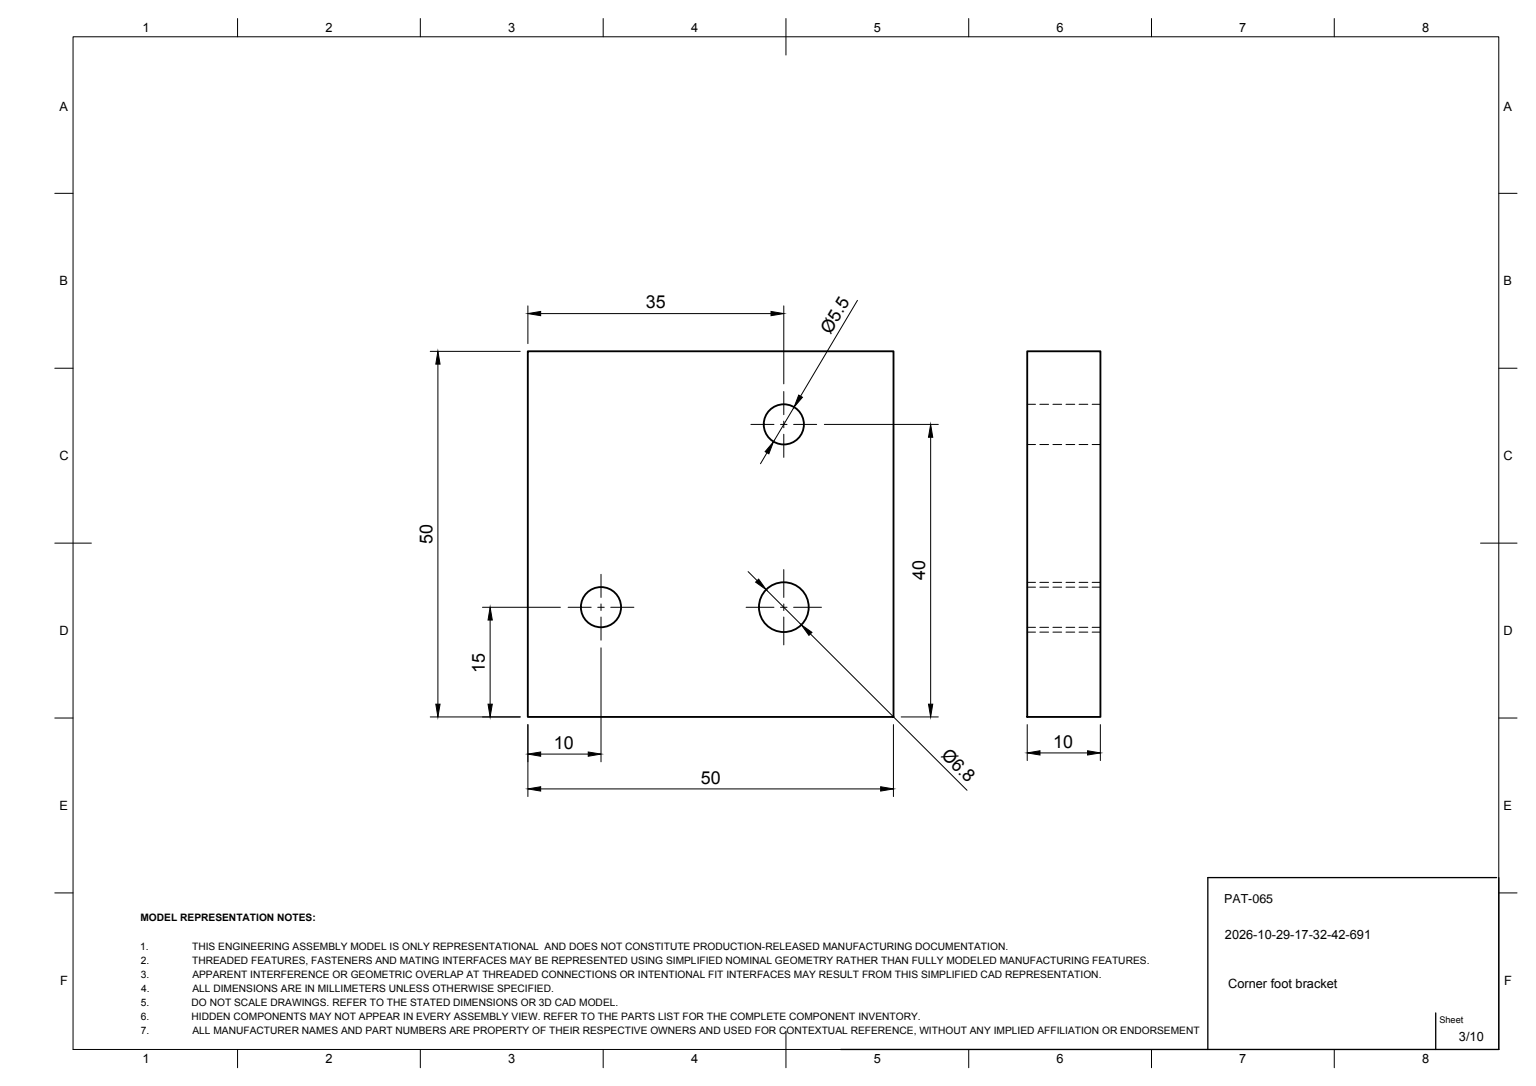
ISO-10303-21;
HEADER;
/* Generated by software containing ST-Developer
 * from STEP Tools, Inc. (www.steptools.com) 
 */

FILE_DESCRIPTION(
/* description */ ('PAT-065'),
/* implementation_level */ '2;1');

FILE_NAME(
/* name */ 'Corner foot bracket.step',
/* time_stamp */ '2026-10-28T22:09:22-07:00',
/* author */ (''),
/* organization */ (''),
/* preprocessor_version */ 'ST-DEVELOPER v20.2',
/* originating_system */ 'Autodesk Translation Framework v15.17.0.0',
/* authorisation */ '');

FILE_SCHEMA (('AUTOMOTIVE_DESIGN { 1 0 10303 214 3 1 1 }'));
ENDSEC;

DATA;
#10=MECHANICAL_DESIGN_GEOMETRIC_PRESENTATION_REPRESENTATION('',(#158),#5502);
#138=SHAPE_REPRESENTATION_RELATIONSHIP('SRR','None',#5555,#148);
#148=ADVANCED_BREP_SHAPE_REPRESENTATION('',(#168),#5491);
#158=STYLED_ITEM('',(#5673),#168);
#168=MANIFOLD_SOLID_BREP('Body1',#3205);
#177=FACE_BOUND('',#519,.T.);
#178=FACE_BOUND('',#520,.T.);
#179=FACE_BOUND('',#521,.T.);
#180=FACE_BOUND('',#523,.T.);
#181=FACE_BOUND('',#524,.T.);
#182=FACE_BOUND('',#525,.T.);
#201=PLANE('',#3338);
#202=PLANE('',#3339);
#203=PLANE('',#3340);
#204=PLANE('',#3341);
#205=PLANE('',#3342);
#206=PLANE('',#3343);
#337=FACE_OUTER_BOUND('',#511,.T.);
#338=FACE_OUTER_BOUND('',#512,.T.);
#339=FACE_OUTER_BOUND('',#513,.T.);
#340=FACE_OUTER_BOUND('',#514,.T.);
#341=FACE_OUTER_BOUND('',#515,.T.);
#342=FACE_OUTER_BOUND('',#516,.T.);
#343=FACE_OUTER_BOUND('',#517,.T.);
#344=FACE_OUTER_BOUND('',#518,.T.);
#345=FACE_OUTER_BOUND('',#522,.T.);
#511=EDGE_LOOP('',(#2152,#2153,#2154,#2155));
#512=EDGE_LOOP('',(#2156,#2157,#2158,#2159));
#513=EDGE_LOOP('',(#2160,#2161,#2162,#2163));
#514=EDGE_LOOP('',(#2164,#2165,#2166,#2167));
#515=EDGE_LOOP('',(#2168,#2169,#2170,#2171));
#516=EDGE_LOOP('',(#2172,#2173,#2174,#2175));
#517=EDGE_LOOP('',(#2176,#2177,#2178,#2179));
#518=EDGE_LOOP('',(#2180,#2181,#2182,#2183));
#519=EDGE_LOOP('',(#2184));
#520=EDGE_LOOP('',(#2185));
#521=EDGE_LOOP('',(#2186));
#522=EDGE_LOOP('',(#2187,#2188,#2189,#2190));
#523=EDGE_LOOP('',(#2191));
#524=EDGE_LOOP('',(#2192));
#525=EDGE_LOOP('',(#2193));
#709=LINE('',#4537,#1040);
#710=LINE('',#4543,#1041);
#711=LINE('',#4549,#1042);
#712=LINE('',#4554,#1043);
#713=LINE('',#4556,#1044);
#714=LINE('',#4558,#1045);
#715=LINE('',#4559,#1046);
#716=LINE('',#4562,#1047);
#717=LINE('',#4564,#1048);
#718=LINE('',#4565,#1049);
#719=LINE('',#4568,#1050);
#720=LINE('',#4570,#1051);
#721=LINE('',#4571,#1052);
#722=LINE('',#4573,#1053);
#723=LINE('',#4574,#1054);
#1040=VECTOR('',#3626,0.275);
#1041=VECTOR('',#3633,0.275);
#1042=VECTOR('',#3640,0.34);
#1043=VECTOR('',#3645,1.);
#1044=VECTOR('',#3646,1.);
#1045=VECTOR('',#3647,1.);
#1046=VECTOR('',#3648,1.);
#1047=VECTOR('',#3651,1.);
#1048=VECTOR('',#3652,1.);
#1049=VECTOR('',#3653,1.);
#1050=VECTOR('',#3656,1.);
#1051=VECTOR('',#3657,1.);
#1052=VECTOR('',#3658,1.);
#1053=VECTOR('',#3661,1.);
#1054=VECTOR('',#3662,1.);
#1371=CIRCLE('',#3330,0.275);
#1372=CIRCLE('',#3331,0.275);
#1373=CIRCLE('',#3333,0.275);
#1374=CIRCLE('',#3334,0.275);
#1375=CIRCLE('',#3336,0.34);
#1376=CIRCLE('',#3337,0.34);
#1444=VERTEX_POINT('',#4534);
#1445=VERTEX_POINT('',#4536);
#1446=VERTEX_POINT('',#4540);
#1447=VERTEX_POINT('',#4542);
#1448=VERTEX_POINT('',#4546);
#1449=VERTEX_POINT('',#4548);
#1450=VERTEX_POINT('',#4552);
#1451=VERTEX_POINT('',#4553);
#1452=VERTEX_POINT('',#4555);
#1453=VERTEX_POINT('',#4557);
#1454=VERTEX_POINT('',#4561);
#1455=VERTEX_POINT('',#4563);
#1456=VERTEX_POINT('',#4567);
#1457=VERTEX_POINT('',#4569);
#1726=EDGE_CURVE('',#1444,#1444,#1371,.T.);
#1727=EDGE_CURVE('',#1444,#1445,#709,.T.);
#1728=EDGE_CURVE('',#1445,#1445,#1372,.T.);
#1729=EDGE_CURVE('',#1446,#1446,#1373,.T.);
#1730=EDGE_CURVE('',#1446,#1447,#710,.T.);
#1731=EDGE_CURVE('',#1447,#1447,#1374,.T.);
#1732=EDGE_CURVE('',#1448,#1448,#1375,.T.);
#1733=EDGE_CURVE('',#1448,#1449,#711,.T.);
#1734=EDGE_CURVE('',#1449,#1449,#1376,.T.);
#1735=EDGE_CURVE('',#1450,#1451,#712,.T.);
#1736=EDGE_CURVE('',#1451,#1452,#713,.T.);
#1737=EDGE_CURVE('',#1453,#1452,#714,.T.);
#1738=EDGE_CURVE('',#1450,#1453,#715,.T.);
#1739=EDGE_CURVE('',#1454,#1450,#716,.T.);
#1740=EDGE_CURVE('',#1455,#1453,#717,.T.);
#1741=EDGE_CURVE('',#1454,#1455,#718,.T.);
#1742=EDGE_CURVE('',#1456,#1454,#719,.T.);
#1743=EDGE_CURVE('',#1457,#1455,#720,.T.);
#1744=EDGE_CURVE('',#1456,#1457,#721,.T.);
#1745=EDGE_CURVE('',#1451,#1456,#722,.T.);
#1746=EDGE_CURVE('',#1452,#1457,#723,.T.);
#2152=ORIENTED_EDGE('',*,*,#1726,.F.);
#2153=ORIENTED_EDGE('',*,*,#1727,.T.);
#2154=ORIENTED_EDGE('',*,*,#1728,.F.);
#2155=ORIENTED_EDGE('',*,*,#1727,.F.);
#2156=ORIENTED_EDGE('',*,*,#1729,.F.);
#2157=ORIENTED_EDGE('',*,*,#1730,.T.);
#2158=ORIENTED_EDGE('',*,*,#1731,.F.);
#2159=ORIENTED_EDGE('',*,*,#1730,.F.);
#2160=ORIENTED_EDGE('',*,*,#1732,.F.);
#2161=ORIENTED_EDGE('',*,*,#1733,.T.);
#2162=ORIENTED_EDGE('',*,*,#1734,.F.);
#2163=ORIENTED_EDGE('',*,*,#1733,.F.);
#2164=ORIENTED_EDGE('',*,*,#1735,.T.);
#2165=ORIENTED_EDGE('',*,*,#1736,.T.);
#2166=ORIENTED_EDGE('',*,*,#1737,.F.);
#2167=ORIENTED_EDGE('',*,*,#1738,.F.);
#2168=ORIENTED_EDGE('',*,*,#1739,.T.);
#2169=ORIENTED_EDGE('',*,*,#1738,.T.);
#2170=ORIENTED_EDGE('',*,*,#1740,.F.);
#2171=ORIENTED_EDGE('',*,*,#1741,.F.);
#2172=ORIENTED_EDGE('',*,*,#1742,.T.);
#2173=ORIENTED_EDGE('',*,*,#1741,.T.);
#2174=ORIENTED_EDGE('',*,*,#1743,.F.);
#2175=ORIENTED_EDGE('',*,*,#1744,.F.);
#2176=ORIENTED_EDGE('',*,*,#1745,.T.);
#2177=ORIENTED_EDGE('',*,*,#1744,.T.);
#2178=ORIENTED_EDGE('',*,*,#1746,.F.);
#2179=ORIENTED_EDGE('',*,*,#1736,.F.);
#2180=ORIENTED_EDGE('',*,*,#1746,.T.);
#2181=ORIENTED_EDGE('',*,*,#1743,.T.);
#2182=ORIENTED_EDGE('',*,*,#1740,.T.);
#2183=ORIENTED_EDGE('',*,*,#1737,.T.);
#2184=ORIENTED_EDGE('',*,*,#1728,.T.);
#2185=ORIENTED_EDGE('',*,*,#1731,.T.);
#2186=ORIENTED_EDGE('',*,*,#1734,.T.);
#2187=ORIENTED_EDGE('',*,*,#1745,.F.);
#2188=ORIENTED_EDGE('',*,*,#1735,.F.);
#2189=ORIENTED_EDGE('',*,*,#1739,.F.);
#2190=ORIENTED_EDGE('',*,*,#1742,.F.);
#2191=ORIENTED_EDGE('',*,*,#1726,.T.);
#2192=ORIENTED_EDGE('',*,*,#1729,.T.);
#2193=ORIENTED_EDGE('',*,*,#1732,.T.);
#3004=CYLINDRICAL_SURFACE('',#3329,0.275);
#3005=CYLINDRICAL_SURFACE('',#3332,0.275);
#3006=CYLINDRICAL_SURFACE('',#3335,0.34);
#3031=ADVANCED_FACE('',(#337),#3004,.F.);
#3032=ADVANCED_FACE('',(#338),#3005,.F.);
#3033=ADVANCED_FACE('',(#339),#3006,.F.);
#3034=ADVANCED_FACE('',(#340),#201,.T.);
#3035=ADVANCED_FACE('',(#341),#202,.T.);
#3036=ADVANCED_FACE('',(#342),#203,.T.);
#3037=ADVANCED_FACE('',(#343),#204,.T.);
#3038=ADVANCED_FACE('',(#344,#177,#178,#179),#205,.T.);
#3039=ADVANCED_FACE('',(#345,#180,#181,#182),#206,.F.);
#3205=CLOSED_SHELL('',(#3031,#3032,#3033,#3034,#3035,#3036,#3037,#3038,
#3039));
#3328=AXIS2_PLACEMENT_3D('',#4532,#3620,#3621);
#3329=AXIS2_PLACEMENT_3D('',#4533,#3622,#3623);
#3330=AXIS2_PLACEMENT_3D('',#4535,#3624,#3625);
#3331=AXIS2_PLACEMENT_3D('',#4538,#3627,#3628);
#3332=AXIS2_PLACEMENT_3D('',#4539,#3629,#3630);
#3333=AXIS2_PLACEMENT_3D('',#4541,#3631,#3632);
#3334=AXIS2_PLACEMENT_3D('',#4544,#3634,#3635);
#3335=AXIS2_PLACEMENT_3D('',#4545,#3636,#3637);
#3336=AXIS2_PLACEMENT_3D('',#4547,#3638,#3639);
#3337=AXIS2_PLACEMENT_3D('',#4550,#3641,#3642);
#3338=AXIS2_PLACEMENT_3D('',#4551,#3643,#3644);
#3339=AXIS2_PLACEMENT_3D('',#4560,#3649,#3650);
#3340=AXIS2_PLACEMENT_3D('',#4566,#3654,#3655);
#3341=AXIS2_PLACEMENT_3D('',#4572,#3659,#3660);
#3342=AXIS2_PLACEMENT_3D('',#4575,#3663,#3664);
#3343=AXIS2_PLACEMENT_3D('',#4576,#3665,#3666);
#3620=DIRECTION('axis',(0.,0.,1.));
#3621=DIRECTION('refdir',(1.,0.,0.));
#3622=DIRECTION('center_axis',(0.,0.,1.));
#3623=DIRECTION('ref_axis',(1.,0.,0.));
#3624=DIRECTION('center_axis',(0.,0.,1.));
#3625=DIRECTION('ref_axis',(1.,0.,0.));
#3626=DIRECTION('',(0.,0.,1.));
#3627=DIRECTION('center_axis',(0.,0.,-1.));
#3628=DIRECTION('ref_axis',(1.,0.,0.));
#3629=DIRECTION('center_axis',(0.,0.,1.));
#3630=DIRECTION('ref_axis',(1.,0.,0.));
#3631=DIRECTION('center_axis',(0.,0.,1.));
#3632=DIRECTION('ref_axis',(1.,0.,0.));
#3633=DIRECTION('',(0.,0.,1.));
#3634=DIRECTION('center_axis',(0.,0.,-1.));
#3635=DIRECTION('ref_axis',(1.,0.,0.));
#3636=DIRECTION('center_axis',(0.,0.,1.));
#3637=DIRECTION('ref_axis',(1.,0.,0.));
#3638=DIRECTION('center_axis',(0.,0.,1.));
#3639=DIRECTION('ref_axis',(1.,0.,0.));
#3640=DIRECTION('',(0.,0.,1.));
#3641=DIRECTION('center_axis',(0.,0.,-1.));
#3642=DIRECTION('ref_axis',(1.,0.,0.));
#3643=DIRECTION('center_axis',(0.,1.,0.));
#3644=DIRECTION('ref_axis',(-1.,0.,0.));
#3645=DIRECTION('',(-1.,0.,0.));
#3646=DIRECTION('',(0.,0.,1.));
#3647=DIRECTION('',(-1.,0.,0.));
#3648=DIRECTION('',(0.,0.,1.));
#3649=DIRECTION('center_axis',(1.,0.,0.));
#3650=DIRECTION('ref_axis',(0.,1.,0.));
#3651=DIRECTION('',(0.,1.,0.));
#3652=DIRECTION('',(0.,1.,0.));
#3653=DIRECTION('',(0.,0.,1.));
#3654=DIRECTION('center_axis',(0.,-1.,0.));
#3655=DIRECTION('ref_axis',(1.,0.,0.));
#3656=DIRECTION('',(1.,0.,0.));
#3657=DIRECTION('',(1.,0.,0.));
#3658=DIRECTION('',(0.,0.,1.));
#3659=DIRECTION('center_axis',(-1.,0.,0.));
#3660=DIRECTION('ref_axis',(0.,-1.,0.));
#3661=DIRECTION('',(0.,-1.,0.));
#3662=DIRECTION('',(0.,-1.,0.));
#3663=DIRECTION('center_axis',(0.,0.,1.));
#3664=DIRECTION('ref_axis',(1.,0.,0.));
#3665=DIRECTION('center_axis',(0.,0.,1.));
#3666=DIRECTION('ref_axis',(1.,0.,0.));
#4532=CARTESIAN_POINT('',(0.,0.,0.));
#4533=CARTESIAN_POINT('Origin',(0.,2.5,4.9));
#4534=CARTESIAN_POINT('',(-0.275,2.5,5.));
#4535=CARTESIAN_POINT('Origin',(0.,2.5,5.));
#4536=CARTESIAN_POINT('',(-0.275,2.5,6.));
#4537=CARTESIAN_POINT('',(-0.275,2.5,4.9));
#4538=CARTESIAN_POINT('Origin',(0.,2.5,6.));
#4539=CARTESIAN_POINT('Origin',(2.5,0.,4.9));
#4540=CARTESIAN_POINT('',(2.225,-3.36777869765522E-17,5.));
#4541=CARTESIAN_POINT('Origin',(2.5,0.,5.));
#4542=CARTESIAN_POINT('',(2.225,3.36777869765522E-17,6.));
#4543=CARTESIAN_POINT('',(2.225,-3.36777869765522E-17,4.9));
#4544=CARTESIAN_POINT('Origin',(2.5,0.,6.));
#4545=CARTESIAN_POINT('Origin',(0.,0.,4.9));
#4546=CARTESIAN_POINT('',(-0.34,-4.163799117101E-17,5.));
#4547=CARTESIAN_POINT('Origin',(0.,0.,5.));
#4548=CARTESIAN_POINT('',(-0.34,4.163799117101E-17,6.));
#4549=CARTESIAN_POINT('',(-0.34,-4.163799117101E-17,4.9));
#4550=CARTESIAN_POINT('Origin',(0.,0.,6.));
#4551=CARTESIAN_POINT('Origin',(3.5,3.5,5.));
#4552=CARTESIAN_POINT('',(3.5,3.5,5.));
#4553=CARTESIAN_POINT('',(-1.5,3.5,5.));
#4554=CARTESIAN_POINT('',(3.5,3.5,5.));
#4555=CARTESIAN_POINT('',(-1.5,3.5,6.));
#4556=CARTESIAN_POINT('',(-1.5,3.5,5.));
#4557=CARTESIAN_POINT('',(3.5,3.5,6.));
#4558=CARTESIAN_POINT('',(3.5,3.5,6.));
#4559=CARTESIAN_POINT('',(3.5,3.5,5.));
#4560=CARTESIAN_POINT('Origin',(3.5,-1.5,5.));
#4561=CARTESIAN_POINT('',(3.5,-1.5,5.));
#4562=CARTESIAN_POINT('',(3.5,-1.5,5.));
#4563=CARTESIAN_POINT('',(3.5,-1.5,6.));
#4564=CARTESIAN_POINT('',(3.5,-1.5,6.));
#4565=CARTESIAN_POINT('',(3.5,-1.5,5.));
#4566=CARTESIAN_POINT('Origin',(-1.5,-1.5,5.));
#4567=CARTESIAN_POINT('',(-1.5,-1.5,5.));
#4568=CARTESIAN_POINT('',(-1.5,-1.5,5.));
#4569=CARTESIAN_POINT('',(-1.5,-1.5,6.));
#4570=CARTESIAN_POINT('',(-1.5,-1.5,6.));
#4571=CARTESIAN_POINT('',(-1.5,-1.5,5.));
#4572=CARTESIAN_POINT('Origin',(-1.5,3.5,5.));
#4573=CARTESIAN_POINT('',(-1.5,3.5,5.));
#4574=CARTESIAN_POINT('',(-1.5,3.5,6.));
#4575=CARTESIAN_POINT('Origin',(1.,1.,6.));
#4576=CARTESIAN_POINT('Origin',(1.,1.,5.));
#5478=UNCERTAINTY_MEASURE_WITH_UNIT(LENGTH_MEASURE(0.001),#5503,
'DISTANCE_ACCURACY_VALUE',
'Maximum model space distance between geometric entities at asserted c
onnectivities');
#5489=UNCERTAINTY_MEASURE_WITH_UNIT(LENGTH_MEASURE(0.001),#5503,
'DISTANCE_ACCURACY_VALUE',
'Maximum model space distance between geometric entities at asserted c
onnectivities');
#5491=(
GEOMETRIC_REPRESENTATION_CONTEXT(3)
GLOBAL_UNCERTAINTY_ASSIGNED_CONTEXT((#5478))
GLOBAL_UNIT_ASSIGNED_CONTEXT((#5503,#5505,#5506))
REPRESENTATION_CONTEXT('','3D')
);
#5502=(
GEOMETRIC_REPRESENTATION_CONTEXT(3)
GLOBAL_UNCERTAINTY_ASSIGNED_CONTEXT((#5489))
GLOBAL_UNIT_ASSIGNED_CONTEXT((#5503,#5505,#5506))
REPRESENTATION_CONTEXT('','3D')
);
#5503=(
LENGTH_UNIT()
NAMED_UNIT(*)
SI_UNIT(.CENTI.,.METRE.)
);
#5505=(
NAMED_UNIT(*)
PLANE_ANGLE_UNIT()
SI_UNIT($,.RADIAN.)
);
#5506=(
NAMED_UNIT(*)
SI_UNIT($,.STERADIAN.)
SOLID_ANGLE_UNIT()
);
#5508=SHAPE_DEFINITION_REPRESENTATION(#5520,#5555);
#5520=PRODUCT_DEFINITION_SHAPE('',$,#5568);
#5555=SHAPE_REPRESENTATION('',(#3328),#5491);
#5566=PRODUCT_DEFINITION_CONTEXT('part definition',#5604,'design');
#5568=PRODUCT_DEFINITION('Corner foot bracket',
'Corner foot bracket',#5580,#5566);
#5580=PRODUCT_DEFINITION_FORMATION('',$,#5607);
#5604=APPLICATION_CONTEXT(
'Core Data for Automotive Mechanical Design Process');
#5605=PRODUCT_CONTEXT('part definition',#5604,'mechanical');
#5607=PRODUCT('Corner foot bracket','Corner foot bracket',
'Corner foot bracket',(#5605));
#5667=COLOUR_RGB('Dark Blue',0.08,0.2,0.34);
#5668=FILL_AREA_STYLE_COLOUR('',#5667);
#5669=FILL_AREA_STYLE('',(#5668));
#5670=SURFACE_STYLE_FILL_AREA(#5669);
#5671=SURFACE_SIDE_STYLE('',(#5670));
#5672=SURFACE_STYLE_USAGE(.BOTH.,#5671);
#5673=PRESENTATION_STYLE_ASSIGNMENT((#5672));
ENDSEC;
END-ISO-10303-21;
